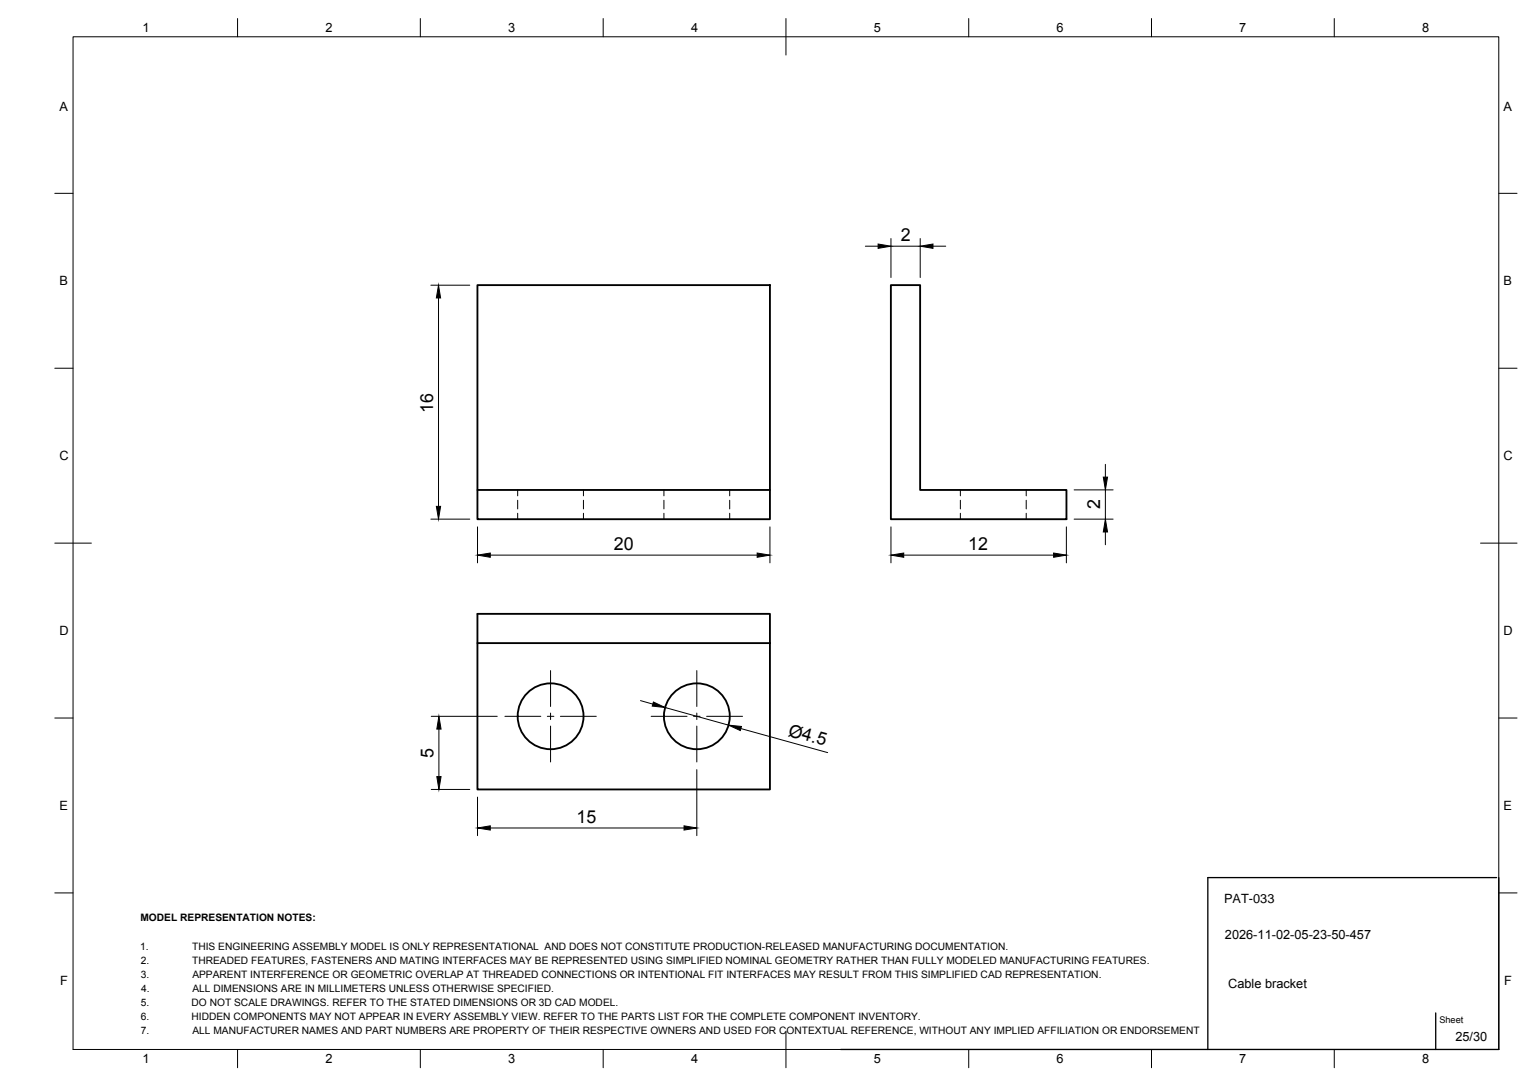
ISO-10303-21;
HEADER;
/* Generated by software containing ST-Developer
 * from STEP Tools, Inc. (www.steptools.com) 
 */

FILE_DESCRIPTION(
/* description */ ('Dual-rail gantry carriage'),
/* implementation_level */ '2;1');

FILE_NAME(
/* name */ 'Cable bracket.step',
/* time_stamp */ '2026-10-27T10:49:15-07:00',
/* author */ (''),
/* organization */ (''),
/* preprocessor_version */ 'ST-DEVELOPER v20.2',
/* originating_system */ 'Autodesk Translation Framework v15.17.0.0',
/* authorisation */ '');

FILE_SCHEMA (('AUTOMOTIVE_DESIGN { 1 0 10303 214 3 1 1 }'));
ENDSEC;

DATA;
#10=MECHANICAL_DESIGN_GEOMETRIC_PRESENTATION_REPRESENTATION('',(#606),#12804);
#544=SHAPE_REPRESENTATION_RELATIONSHIP('SRR','None',#13023,#575);
#575=ADVANCED_BREP_SHAPE_REPRESENTATION('',(#635),#12793);
#606=STYLED_ITEM('',(#13226),#635);
#635=MANIFOLD_SOLID_BREP('Body1',#7386);
#747=FACE_BOUND('',#1818,.T.);
#748=FACE_BOUND('',#1819,.T.);
#749=FACE_BOUND('',#1824,.T.);
#750=FACE_BOUND('',#1825,.T.);
#963=PLANE('',#8190);
#964=PLANE('',#8191);
#965=PLANE('',#8192);
#966=PLANE('',#8193);
#967=PLANE('',#8194);
#968=PLANE('',#8195);
#969=PLANE('',#8196);
#970=PLANE('',#8197);
#1321=FACE_OUTER_BOUND('',#1815,.T.);
#1322=FACE_OUTER_BOUND('',#1816,.T.);
#1323=FACE_OUTER_BOUND('',#1817,.T.);
#1324=FACE_OUTER_BOUND('',#1820,.T.);
#1325=FACE_OUTER_BOUND('',#1821,.T.);
#1326=FACE_OUTER_BOUND('',#1822,.T.);
#1327=FACE_OUTER_BOUND('',#1823,.T.);
#1328=FACE_OUTER_BOUND('',#1826,.T.);
#1329=FACE_OUTER_BOUND('',#1827,.T.);
#1330=FACE_OUTER_BOUND('',#1828,.T.);
#1815=EDGE_LOOP('',(#6369,#6370,#6371,#6372));
#1816=EDGE_LOOP('',(#6373,#6374,#6375,#6376));
#1817=EDGE_LOOP('',(#6377,#6378,#6379,#6380));
#1818=EDGE_LOOP('',(#6381));
#1819=EDGE_LOOP('',(#6382));
#1820=EDGE_LOOP('',(#6383,#6384,#6385,#6386));
#1821=EDGE_LOOP('',(#6387,#6388,#6389,#6390));
#1822=EDGE_LOOP('',(#6391,#6392,#6393,#6394));
#1823=EDGE_LOOP('',(#6395,#6396,#6397,#6398));
#1824=EDGE_LOOP('',(#6399));
#1825=EDGE_LOOP('',(#6400));
#1826=EDGE_LOOP('',(#6401,#6402,#6403,#6404));
#1827=EDGE_LOOP('',(#6405,#6406,#6407,#6408,#6409,#6410));
#1828=EDGE_LOOP('',(#6411,#6412,#6413,#6414,#6415,#6416));
#2454=LINE('',#12062,#3163);
#2455=LINE('',#12068,#3164);
#2456=LINE('',#12073,#3165);
#2457=LINE('',#12075,#3166);
#2458=LINE('',#12077,#3167);
#2459=LINE('',#12078,#3168);
#2460=LINE('',#12081,#3169);
#2461=LINE('',#12083,#3170);
#2462=LINE('',#12084,#3171);
#2463=LINE('',#12087,#3172);
#2464=LINE('',#12089,#3173);
#2465=LINE('',#12090,#3174);
#2466=LINE('',#12093,#3175);
#2467=LINE('',#12095,#3176);
#2468=LINE('',#12096,#3177);
#2469=LINE('',#12099,#3178);
#2470=LINE('',#12101,#3179);
#2471=LINE('',#12102,#3180);
#2472=LINE('',#12104,#3181);
#2473=LINE('',#12105,#3182);
#3163=VECTOR('',#9883,0.225000000000001);
#3164=VECTOR('',#9890,0.225000000000001);
#3165=VECTOR('',#9895,1.);
#3166=VECTOR('',#9896,1.);
#3167=VECTOR('',#9897,1.);
#3168=VECTOR('',#9898,1.);
#3169=VECTOR('',#9901,1.);
#3170=VECTOR('',#9902,1.);
#3171=VECTOR('',#9903,1.);
#3172=VECTOR('',#9906,1.);
#3173=VECTOR('',#9907,1.);
#3174=VECTOR('',#9908,1.);
#3175=VECTOR('',#9911,1.);
#3176=VECTOR('',#9912,1.);
#3177=VECTOR('',#9913,1.);
#3178=VECTOR('',#9916,1.);
#3179=VECTOR('',#9917,1.);
#3180=VECTOR('',#9918,1.);
#3181=VECTOR('',#9921,1.);
#3182=VECTOR('',#9922,1.);
#3509=CIRCLE('',#8185,0.225000000000001);
#3510=CIRCLE('',#8186,0.225000000000001);
#3511=CIRCLE('',#8188,0.225000000000001);
#3512=CIRCLE('',#8189,0.225000000000001);
#3987=VERTEX_POINT('',#12059);
#3988=VERTEX_POINT('',#12061);
#3989=VERTEX_POINT('',#12065);
#3990=VERTEX_POINT('',#12067);
#3991=VERTEX_POINT('',#12071);
#3992=VERTEX_POINT('',#12072);
#3993=VERTEX_POINT('',#12074);
#3994=VERTEX_POINT('',#12076);
#3995=VERTEX_POINT('',#12080);
#3996=VERTEX_POINT('',#12082);
#3997=VERTEX_POINT('',#12086);
#3998=VERTEX_POINT('',#12088);
#3999=VERTEX_POINT('',#12092);
#4000=VERTEX_POINT('',#12094);
#4001=VERTEX_POINT('',#12098);
#4002=VERTEX_POINT('',#12100);
#4807=EDGE_CURVE('',#3987,#3987,#3509,.T.);
#4808=EDGE_CURVE('',#3987,#3988,#2454,.T.);
#4809=EDGE_CURVE('',#3988,#3988,#3510,.T.);
#4810=EDGE_CURVE('',#3989,#3989,#3511,.T.);
#4811=EDGE_CURVE('',#3989,#3990,#2455,.T.);
#4812=EDGE_CURVE('',#3990,#3990,#3512,.T.);
#4813=EDGE_CURVE('',#3991,#3992,#2456,.T.);
#4814=EDGE_CURVE('',#3992,#3993,#2457,.T.);
#4815=EDGE_CURVE('',#3994,#3993,#2458,.T.);
#4816=EDGE_CURVE('',#3991,#3994,#2459,.T.);
#4817=EDGE_CURVE('',#3995,#3991,#2460,.T.);
#4818=EDGE_CURVE('',#3996,#3994,#2461,.T.);
#4819=EDGE_CURVE('',#3995,#3996,#2462,.T.);
#4820=EDGE_CURVE('',#3997,#3995,#2463,.T.);
#4821=EDGE_CURVE('',#3998,#3996,#2464,.T.);
#4822=EDGE_CURVE('',#3997,#3998,#2465,.T.);
#4823=EDGE_CURVE('',#3999,#3997,#2466,.T.);
#4824=EDGE_CURVE('',#4000,#3998,#2467,.T.);
#4825=EDGE_CURVE('',#3999,#4000,#2468,.T.);
#4826=EDGE_CURVE('',#4001,#3999,#2469,.T.);
#4827=EDGE_CURVE('',#4002,#4000,#2470,.T.);
#4828=EDGE_CURVE('',#4001,#4002,#2471,.T.);
#4829=EDGE_CURVE('',#3992,#4001,#2472,.T.);
#4830=EDGE_CURVE('',#3993,#4002,#2473,.T.);
#6369=ORIENTED_EDGE('',*,*,#4807,.F.);
#6370=ORIENTED_EDGE('',*,*,#4808,.T.);
#6371=ORIENTED_EDGE('',*,*,#4809,.F.);
#6372=ORIENTED_EDGE('',*,*,#4808,.F.);
#6373=ORIENTED_EDGE('',*,*,#4810,.F.);
#6374=ORIENTED_EDGE('',*,*,#4811,.T.);
#6375=ORIENTED_EDGE('',*,*,#4812,.F.);
#6376=ORIENTED_EDGE('',*,*,#4811,.F.);
#6377=ORIENTED_EDGE('',*,*,#4813,.T.);
#6378=ORIENTED_EDGE('',*,*,#4814,.T.);
#6379=ORIENTED_EDGE('',*,*,#4815,.F.);
#6380=ORIENTED_EDGE('',*,*,#4816,.F.);
#6381=ORIENTED_EDGE('',*,*,#4809,.T.);
#6382=ORIENTED_EDGE('',*,*,#4812,.T.);
#6383=ORIENTED_EDGE('',*,*,#4817,.T.);
#6384=ORIENTED_EDGE('',*,*,#4816,.T.);
#6385=ORIENTED_EDGE('',*,*,#4818,.F.);
#6386=ORIENTED_EDGE('',*,*,#4819,.F.);
#6387=ORIENTED_EDGE('',*,*,#4820,.T.);
#6388=ORIENTED_EDGE('',*,*,#4819,.T.);
#6389=ORIENTED_EDGE('',*,*,#4821,.F.);
#6390=ORIENTED_EDGE('',*,*,#4822,.F.);
#6391=ORIENTED_EDGE('',*,*,#4823,.T.);
#6392=ORIENTED_EDGE('',*,*,#4822,.T.);
#6393=ORIENTED_EDGE('',*,*,#4824,.F.);
#6394=ORIENTED_EDGE('',*,*,#4825,.F.);
#6395=ORIENTED_EDGE('',*,*,#4826,.T.);
#6396=ORIENTED_EDGE('',*,*,#4825,.T.);
#6397=ORIENTED_EDGE('',*,*,#4827,.F.);
#6398=ORIENTED_EDGE('',*,*,#4828,.F.);
#6399=ORIENTED_EDGE('',*,*,#4807,.T.);
#6400=ORIENTED_EDGE('',*,*,#4810,.T.);
#6401=ORIENTED_EDGE('',*,*,#4829,.T.);
#6402=ORIENTED_EDGE('',*,*,#4828,.T.);
#6403=ORIENTED_EDGE('',*,*,#4830,.F.);
#6404=ORIENTED_EDGE('',*,*,#4814,.F.);
#6405=ORIENTED_EDGE('',*,*,#4830,.T.);
#6406=ORIENTED_EDGE('',*,*,#4827,.T.);
#6407=ORIENTED_EDGE('',*,*,#4824,.T.);
#6408=ORIENTED_EDGE('',*,*,#4821,.T.);
#6409=ORIENTED_EDGE('',*,*,#4818,.T.);
#6410=ORIENTED_EDGE('',*,*,#4815,.T.);
#6411=ORIENTED_EDGE('',*,*,#4829,.F.);
#6412=ORIENTED_EDGE('',*,*,#4813,.F.);
#6413=ORIENTED_EDGE('',*,*,#4817,.F.);
#6414=ORIENTED_EDGE('',*,*,#4820,.F.);
#6415=ORIENTED_EDGE('',*,*,#4823,.F.);
#6416=ORIENTED_EDGE('',*,*,#4826,.F.);
#6956=CYLINDRICAL_SURFACE('',#8184,0.225000000000001);
#6957=CYLINDRICAL_SURFACE('',#8187,0.225000000000001);
#7247=ADVANCED_FACE('',(#1321),#6956,.F.);
#7248=ADVANCED_FACE('',(#1322),#6957,.F.);
#7249=ADVANCED_FACE('',(#1323,#747,#748),#963,.T.);
#7250=ADVANCED_FACE('',(#1324),#964,.T.);
#7251=ADVANCED_FACE('',(#1325),#965,.T.);
#7252=ADVANCED_FACE('',(#1326),#966,.T.);
#7253=ADVANCED_FACE('',(#1327,#749,#750),#967,.T.);
#7254=ADVANCED_FACE('',(#1328),#968,.T.);
#7255=ADVANCED_FACE('',(#1329),#969,.T.);
#7256=ADVANCED_FACE('',(#1330),#970,.F.);
#7386=CLOSED_SHELL('',(#7247,#7248,#7249,#7250,#7251,#7252,#7253,#7254,
#7255,#7256));
#8183=AXIS2_PLACEMENT_3D('',#12057,#9877,#9878);
#8184=AXIS2_PLACEMENT_3D('',#12058,#9879,#9880);
#8185=AXIS2_PLACEMENT_3D('',#12060,#9881,#9882);
#8186=AXIS2_PLACEMENT_3D('',#12063,#9884,#9885);
#8187=AXIS2_PLACEMENT_3D('',#12064,#9886,#9887);
#8188=AXIS2_PLACEMENT_3D('',#12066,#9888,#9889);
#8189=AXIS2_PLACEMENT_3D('',#12069,#9891,#9892);
#8190=AXIS2_PLACEMENT_3D('',#12070,#9893,#9894);
#8191=AXIS2_PLACEMENT_3D('',#12079,#9899,#9900);
#8192=AXIS2_PLACEMENT_3D('',#12085,#9904,#9905);
#8193=AXIS2_PLACEMENT_3D('',#12091,#9909,#9910);
#8194=AXIS2_PLACEMENT_3D('',#12097,#9914,#9915);
#8195=AXIS2_PLACEMENT_3D('',#12103,#9919,#9920);
#8196=AXIS2_PLACEMENT_3D('',#12106,#9923,#9924);
#8197=AXIS2_PLACEMENT_3D('',#12107,#9925,#9926);
#9877=DIRECTION('axis',(0.,0.,1.));
#9878=DIRECTION('refdir',(1.,0.,0.));
#9879=DIRECTION('center_axis',(0.,0.,1.));
#9880=DIRECTION('ref_axis',(1.,0.,0.));
#9881=DIRECTION('center_axis',(0.,0.,1.));
#9882=DIRECTION('ref_axis',(1.,0.,0.));
#9883=DIRECTION('',(0.,0.,1.));
#9884=DIRECTION('center_axis',(0.,0.,-1.));
#9885=DIRECTION('ref_axis',(1.,0.,0.));
#9886=DIRECTION('center_axis',(0.,0.,1.));
#9887=DIRECTION('ref_axis',(1.,0.,0.));
#9888=DIRECTION('center_axis',(0.,0.,1.));
#9889=DIRECTION('ref_axis',(1.,0.,0.));
#9890=DIRECTION('',(0.,0.,1.));
#9891=DIRECTION('center_axis',(0.,0.,-1.));
#9892=DIRECTION('ref_axis',(1.,0.,0.));
#9893=DIRECTION('center_axis',(0.,0.,1.));
#9894=DIRECTION('ref_axis',(0.,-1.,0.));
#9895=DIRECTION('',(0.,-1.,0.));
#9896=DIRECTION('',(1.,0.,0.));
#9897=DIRECTION('',(0.,-1.,0.));
#9898=DIRECTION('',(1.,0.,0.));
#9899=DIRECTION('center_axis',(0.,-1.,0.));
#9900=DIRECTION('ref_axis',(0.,0.,-1.));
#9901=DIRECTION('',(0.,0.,-1.));
#9902=DIRECTION('',(0.,0.,-1.));
#9903=DIRECTION('',(1.,0.,0.));
#9904=DIRECTION('center_axis',(0.,0.,1.));
#9905=DIRECTION('ref_axis',(0.,-1.,0.));
#9906=DIRECTION('',(0.,-1.,0.));
#9907=DIRECTION('',(0.,-1.,0.));
#9908=DIRECTION('',(1.,0.,0.));
#9909=DIRECTION('center_axis',(0.,1.,0.));
#9910=DIRECTION('ref_axis',(0.,0.,1.));
#9911=DIRECTION('',(0.,0.,1.));
#9912=DIRECTION('',(0.,0.,1.));
#9913=DIRECTION('',(1.,0.,0.));
#9914=DIRECTION('center_axis',(0.,0.,-1.));
#9915=DIRECTION('ref_axis',(0.,1.,0.));
#9916=DIRECTION('',(0.,1.,0.));
#9917=DIRECTION('',(0.,1.,0.));
#9918=DIRECTION('',(1.,0.,0.));
#9919=DIRECTION('center_axis',(0.,-1.,0.));
#9920=DIRECTION('ref_axis',(0.,0.,-1.));
#9921=DIRECTION('',(0.,0.,-1.));
#9922=DIRECTION('',(0.,0.,-1.));
#9923=DIRECTION('center_axis',(1.,0.,0.));
#9924=DIRECTION('ref_axis',(0.,0.,-1.));
#9925=DIRECTION('center_axis',(1.,0.,0.));
#9926=DIRECTION('ref_axis',(0.,0.,-1.));
#12057=CARTESIAN_POINT('',(0.,0.,0.));
#12058=CARTESIAN_POINT('Origin',(19.5,12.5,6.3));
#12059=CARTESIAN_POINT('',(19.275,12.5,6.4));
#12060=CARTESIAN_POINT('Origin',(19.5,12.5,6.4));
#12061=CARTESIAN_POINT('',(19.275,12.5,6.6));
#12062=CARTESIAN_POINT('',(19.275,12.5,6.3));
#12063=CARTESIAN_POINT('Origin',(19.5,12.5,6.6));
#12064=CARTESIAN_POINT('Origin',(20.5,12.5,6.3));
#12065=CARTESIAN_POINT('',(20.275,12.5,6.4));
#12066=CARTESIAN_POINT('Origin',(20.5,12.5,6.4));
#12067=CARTESIAN_POINT('',(20.275,12.5,6.6));
#12068=CARTESIAN_POINT('',(20.275,12.5,6.3));
#12069=CARTESIAN_POINT('Origin',(20.5,12.5,6.6));
#12070=CARTESIAN_POINT('Origin',(19.,13.,6.6));
#12071=CARTESIAN_POINT('',(19.,13.,6.6));
#12072=CARTESIAN_POINT('',(19.,12.,6.6));
#12073=CARTESIAN_POINT('',(19.,13.,6.6));
#12074=CARTESIAN_POINT('',(21.,12.,6.6));
#12075=CARTESIAN_POINT('',(19.,12.,6.6));
#12076=CARTESIAN_POINT('',(21.,13.,6.6));
#12077=CARTESIAN_POINT('',(21.,13.,6.6));
#12078=CARTESIAN_POINT('',(19.,13.,6.6));
#12079=CARTESIAN_POINT('Origin',(19.,13.,8.));
#12080=CARTESIAN_POINT('',(19.,13.,8.));
#12081=CARTESIAN_POINT('',(19.,13.,8.));
#12082=CARTESIAN_POINT('',(21.,13.,8.));
#12083=CARTESIAN_POINT('',(21.,13.,8.));
#12084=CARTESIAN_POINT('',(19.,13.,8.));
#12085=CARTESIAN_POINT('Origin',(19.,13.2,8.));
#12086=CARTESIAN_POINT('',(19.,13.2,8.));
#12087=CARTESIAN_POINT('',(19.,13.2,8.));
#12088=CARTESIAN_POINT('',(21.,13.2,8.));
#12089=CARTESIAN_POINT('',(21.,13.2,8.));
#12090=CARTESIAN_POINT('',(19.,13.2,8.));
#12091=CARTESIAN_POINT('Origin',(19.,13.2,6.4));
#12092=CARTESIAN_POINT('',(19.,13.2,6.4));
#12093=CARTESIAN_POINT('',(19.,13.2,6.4));
#12094=CARTESIAN_POINT('',(21.,13.2,6.4));
#12095=CARTESIAN_POINT('',(21.,13.2,6.4));
#12096=CARTESIAN_POINT('',(19.,13.2,6.4));
#12097=CARTESIAN_POINT('Origin',(19.,12.,6.4));
#12098=CARTESIAN_POINT('',(19.,12.,6.4));
#12099=CARTESIAN_POINT('',(19.,12.,6.4));
#12100=CARTESIAN_POINT('',(21.,12.,6.4));
#12101=CARTESIAN_POINT('',(21.,12.,6.4));
#12102=CARTESIAN_POINT('',(19.,12.,6.4));
#12103=CARTESIAN_POINT('Origin',(19.,12.,6.6));
#12104=CARTESIAN_POINT('',(19.,12.,6.6));
#12105=CARTESIAN_POINT('',(21.,12.,6.6));
#12106=CARTESIAN_POINT('Origin',(21.,12.6,7.2));
#12107=CARTESIAN_POINT('Origin',(19.,12.6,7.2));
#12757=UNCERTAINTY_MEASURE_WITH_UNIT(LENGTH_MEASURE(0.001),#12805,
'DISTANCE_ACCURACY_VALUE',
'Maximum model space distance between geometric entities at asserted c
onnectivities');
#12768=UNCERTAINTY_MEASURE_WITH_UNIT(LENGTH_MEASURE(0.001),#12805,
'DISTANCE_ACCURACY_VALUE',
'Maximum model space distance between geometric entities at asserted c
onnectivities');
#12793=(
GEOMETRIC_REPRESENTATION_CONTEXT(3)
GLOBAL_UNCERTAINTY_ASSIGNED_CONTEXT((#12757))
GLOBAL_UNIT_ASSIGNED_CONTEXT((#12805,#12807,#12808))
REPRESENTATION_CONTEXT('','3D')
);
#12804=(
GEOMETRIC_REPRESENTATION_CONTEXT(3)
GLOBAL_UNCERTAINTY_ASSIGNED_CONTEXT((#12768))
GLOBAL_UNIT_ASSIGNED_CONTEXT((#12805,#12807,#12808))
REPRESENTATION_CONTEXT('','3D')
);
#12805=(
LENGTH_UNIT()
NAMED_UNIT(*)
SI_UNIT(.CENTI.,.METRE.)
);
#12807=(
NAMED_UNIT(*)
PLANE_ANGLE_UNIT()
SI_UNIT($,.RADIAN.)
);
#12808=(
NAMED_UNIT(*)
SI_UNIT($,.STERADIAN.)
SOLID_ANGLE_UNIT()
);
#12833=SHAPE_DEFINITION_REPRESENTATION(#12868,#13023);
#12868=PRODUCT_DEFINITION_SHAPE('',$,#13059);
#13023=SHAPE_REPRESENTATION('',(#8183),#12793);
#13034=PRODUCT_DEFINITION_CONTEXT('part definition',#13141,'design');
#13059=PRODUCT_DEFINITION('Cable bracket','Cable bracket',#13094,#13034);
#13094=PRODUCT_DEFINITION_FORMATION('',$,#13167);
#13141=APPLICATION_CONTEXT(
'Core Data for Automotive Mechanical Design Process');
#13142=PRODUCT_CONTEXT('part definition',#13141,'mechanical');
#13167=PRODUCT('Cable bracket','Cable bracket','Cable bracket',(#13142));
#13220=COLOUR_RGB('Dark Blue',0.08,0.2,0.34);
#13221=FILL_AREA_STYLE_COLOUR('',#13220);
#13222=FILL_AREA_STYLE('',(#13221));
#13223=SURFACE_STYLE_FILL_AREA(#13222);
#13224=SURFACE_SIDE_STYLE('',(#13223));
#13225=SURFACE_STYLE_USAGE(.BOTH.,#13224);
#13226=PRESENTATION_STYLE_ASSIGNMENT((#13225));
ENDSEC;
END-ISO-10303-21;
